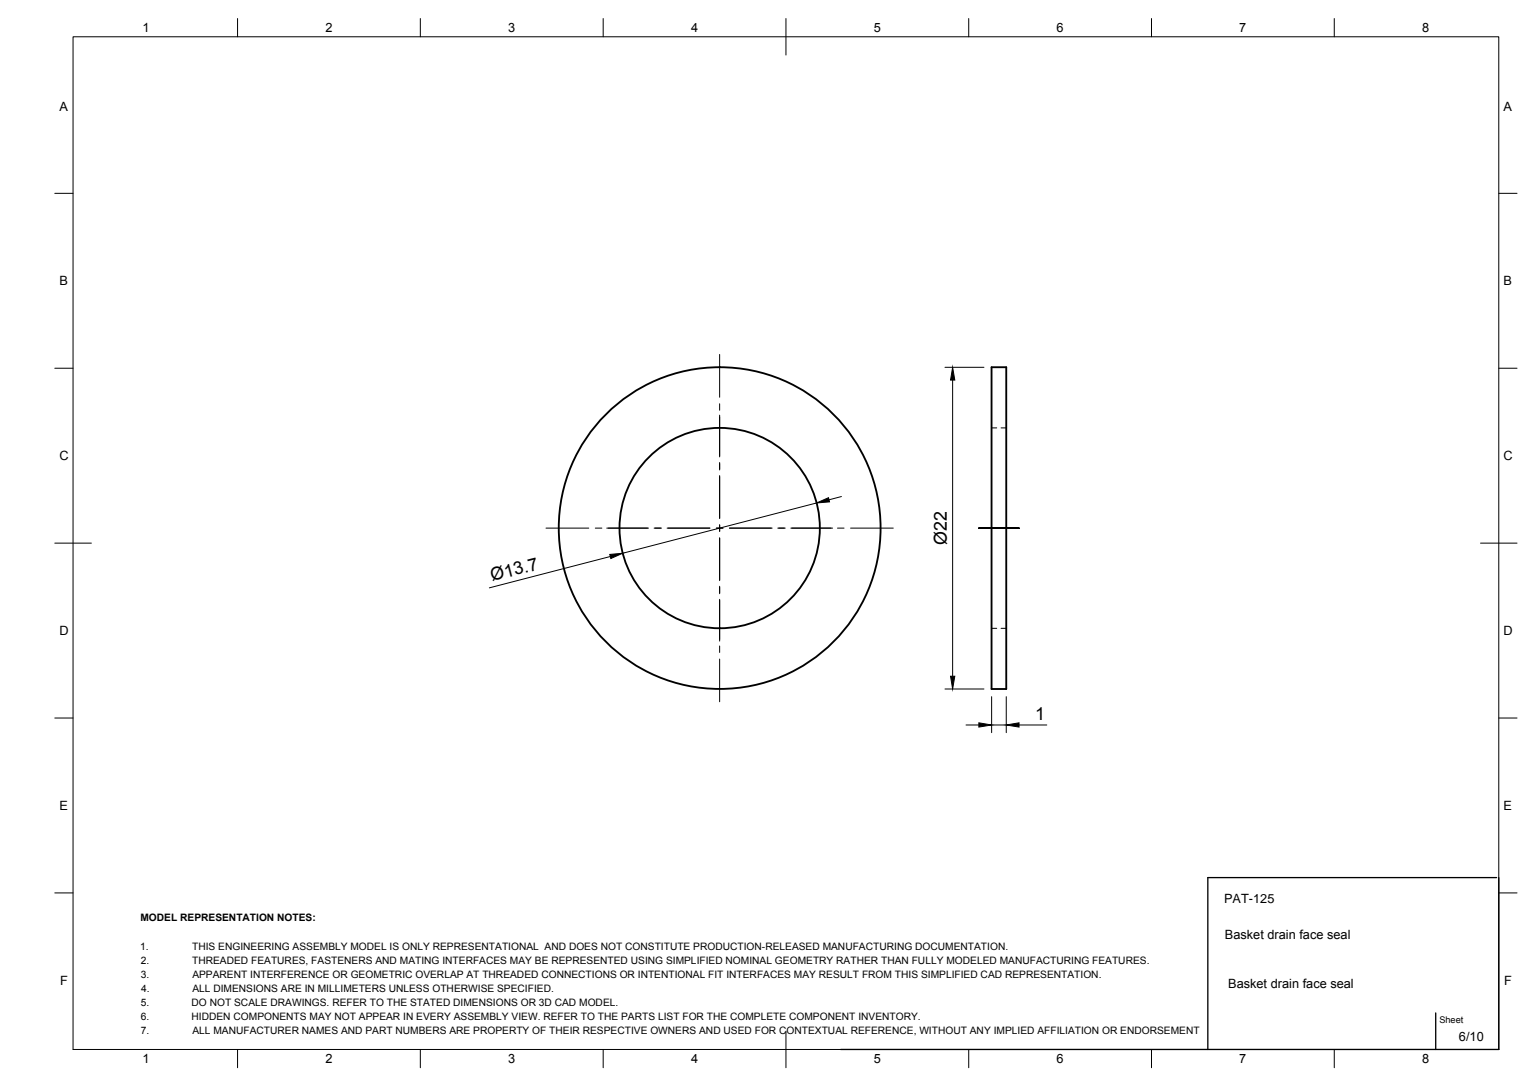
ISO-10303-21;
HEADER;
/* Generated by software containing ST-Developer
 * from STEP Tools, Inc. (www.steptools.com) 
 */

FILE_DESCRIPTION(
/* description */ ('Y-strainer with drain'),
/* implementation_level */ '2;1');

FILE_NAME(
/* name */ 'Basket drain face seal.step',
/* time_stamp */ '2026-10-28T00:41:55-07:00',
/* author */ (''),
/* organization */ (''),
/* preprocessor_version */ 'ST-DEVELOPER v20.2',
/* originating_system */ 'Autodesk Translation Framework v15.17.0.0',
/* authorisation */ '');

FILE_SCHEMA (('AUTOMOTIVE_DESIGN { 1 0 10303 214 3 1 1 }'));
ENDSEC;

DATA;
#10=MECHANICAL_DESIGN_GEOMETRIC_PRESENTATION_REPRESENTATION('',(#96),#8864);
#78=SHAPE_REPRESENTATION_RELATIONSHIP('SRR','None',#8910,#87);
#87=ADVANCED_BREP_SHAPE_REPRESENTATION('',(#105),#8858);
#96=STYLED_ITEM('',(#9040),#105);
#105=MANIFOLD_SOLID_BREP('Body1',#3386);
#427=FACE_BOUND('',#871,.T.);
#428=FACE_BOUND('',#873,.T.);
#483=PLANE('',#3646);
#484=PLANE('',#3647);
#608=FACE_OUTER_BOUND('',#868,.T.);
#609=FACE_OUTER_BOUND('',#869,.T.);
#610=FACE_OUTER_BOUND('',#870,.T.);
#611=FACE_OUTER_BOUND('',#872,.T.);
#868=EDGE_LOOP('',(#2882,#2883,#2884,#2885));
#869=EDGE_LOOP('',(#2886,#2887,#2888,#2889));
#870=EDGE_LOOP('',(#2890));
#871=EDGE_LOOP('',(#2891));
#872=EDGE_LOOP('',(#2892));
#873=EDGE_LOOP('',(#2893));
#1043=LINE('',#8549,#1206);
#1044=LINE('',#8555,#1207);
#1206=VECTOR('',#4151,0.685);
#1207=VECTOR('',#4158,1.1);
#1331=CIRCLE('',#3641,0.685);
#1332=CIRCLE('',#3642,0.685);
#1333=CIRCLE('',#3644,1.1);
#1334=CIRCLE('',#3645,1.1);
#1637=VERTEX_POINT('',#8546);
#1638=VERTEX_POINT('',#8548);
#1639=VERTEX_POINT('',#8552);
#1640=VERTEX_POINT('',#8554);
#2065=EDGE_CURVE('',#1637,#1637,#1331,.T.);
#2066=EDGE_CURVE('',#1637,#1638,#1043,.T.);
#2067=EDGE_CURVE('',#1638,#1638,#1332,.T.);
#2068=EDGE_CURVE('',#1639,#1639,#1333,.T.);
#2069=EDGE_CURVE('',#1639,#1640,#1044,.T.);
#2070=EDGE_CURVE('',#1640,#1640,#1334,.T.);
#2882=ORIENTED_EDGE('',*,*,#2065,.F.);
#2883=ORIENTED_EDGE('',*,*,#2066,.T.);
#2884=ORIENTED_EDGE('',*,*,#2067,.T.);
#2885=ORIENTED_EDGE('',*,*,#2066,.F.);
#2886=ORIENTED_EDGE('',*,*,#2068,.F.);
#2887=ORIENTED_EDGE('',*,*,#2069,.T.);
#2888=ORIENTED_EDGE('',*,*,#2070,.T.);
#2889=ORIENTED_EDGE('',*,*,#2069,.F.);
#2890=ORIENTED_EDGE('',*,*,#2068,.T.);
#2891=ORIENTED_EDGE('',*,*,#2065,.T.);
#2892=ORIENTED_EDGE('',*,*,#2070,.F.);
#2893=ORIENTED_EDGE('',*,*,#2067,.F.);
#3210=CYLINDRICAL_SURFACE('',#3640,0.685);
#3211=CYLINDRICAL_SURFACE('',#3643,1.1);
#3319=ADVANCED_FACE('',(#608),#3210,.F.);
#3320=ADVANCED_FACE('',(#609),#3211,.T.);
#3321=ADVANCED_FACE('',(#610,#427),#483,.T.);
#3322=ADVANCED_FACE('',(#611,#428),#484,.F.);
#3386=CLOSED_SHELL('',(#3319,#3320,#3321,#3322));
#3639=AXIS2_PLACEMENT_3D('',#8544,#4145,#4146);
#3640=AXIS2_PLACEMENT_3D('',#8545,#4147,#4148);
#3641=AXIS2_PLACEMENT_3D('',#8547,#4149,#4150);
#3642=AXIS2_PLACEMENT_3D('',#8550,#4152,#4153);
#3643=AXIS2_PLACEMENT_3D('',#8551,#4154,#4155);
#3644=AXIS2_PLACEMENT_3D('',#8553,#4156,#4157);
#3645=AXIS2_PLACEMENT_3D('',#8556,#4159,#4160);
#3646=AXIS2_PLACEMENT_3D('',#8557,#4161,#4162);
#3647=AXIS2_PLACEMENT_3D('',#8558,#4163,#4164);
#4145=DIRECTION('axis',(0.,0.,1.));
#4146=DIRECTION('refdir',(1.,0.,0.));
#4147=DIRECTION('center_axis',(0.707106781186548,0.,-0.707106781186547));
#4148=DIRECTION('ref_axis',(-0.707106781186547,0.,-0.707106781186548));
#4149=DIRECTION('center_axis',(-0.707106781186548,0.,0.707106781186547));
#4150=DIRECTION('ref_axis',(-0.707106781186547,0.,-0.707106781186548));
#4151=DIRECTION('',(-0.707106781186548,0.,0.707106781186547));
#4152=DIRECTION('center_axis',(-0.707106781186548,0.,0.707106781186547));
#4153=DIRECTION('ref_axis',(-0.707106781186547,0.,-0.707106781186548));
#4154=DIRECTION('center_axis',(0.707106781186548,0.,-0.707106781186547));
#4155=DIRECTION('ref_axis',(-0.707106781186547,0.,-0.707106781186548));
#4156=DIRECTION('center_axis',(0.707106781186548,0.,-0.707106781186547));
#4157=DIRECTION('ref_axis',(-0.707106781186547,0.,-0.707106781186548));
#4158=DIRECTION('',(-0.707106781186548,0.,0.707106781186547));
#4159=DIRECTION('center_axis',(0.707106781186548,0.,-0.707106781186547));
#4160=DIRECTION('ref_axis',(-0.707106781186547,0.,-0.707106781186548));
#4161=DIRECTION('center_axis',(0.707106781186548,0.,-0.707106781186547));
#4162=DIRECTION('ref_axis',(-0.707106781186547,0.,-0.707106781186548));
#4163=DIRECTION('center_axis',(0.707106781186548,0.,-0.707106781186547));
#4164=DIRECTION('ref_axis',(-0.707106781186547,0.,-0.707106781186548));
#8544=CARTESIAN_POINT('',(0.,0.,0.));
#8545=CARTESIAN_POINT('Origin',(3.45477272147525,0.,2.54522727852475));
#8546=CARTESIAN_POINT('',(4.00985154470669,-8.38883057415937E-17,2.95888474551888));
#8547=CARTESIAN_POINT('Origin',(3.5254833995939,0.,2.4745166004061));
#8548=CARTESIAN_POINT('',(3.93914086658804,-8.38883057415937E-17,3.02959542363754));
#8549=CARTESIAN_POINT('',(3.93914086658804,-8.38883057415937E-17,3.02959542363754));
#8550=CARTESIAN_POINT('Origin',(3.45477272147525,0.,2.54522727852475));
#8551=CARTESIAN_POINT('Origin',(3.45477272147525,0.,2.54522727852475));
#8552=CARTESIAN_POINT('',(4.30330085889911,-1.34711147906209E-16,3.2523340597113));
#8553=CARTESIAN_POINT('Origin',(3.5254833995939,0.,2.4745166004061));
#8554=CARTESIAN_POINT('',(4.23259018078045,-1.34711147906209E-16,3.32304473782995));
#8555=CARTESIAN_POINT('',(4.23259018078045,-1.34711147906209E-16,3.32304473782995));
#8556=CARTESIAN_POINT('Origin',(3.45477272147525,0.,2.54522727852475));
#8557=CARTESIAN_POINT('Origin',(3.5254833995939,0.,2.4745166004061));
#8558=CARTESIAN_POINT('Origin',(3.45477272147525,0.,2.54522727852475));
#8846=UNCERTAINTY_MEASURE_WITH_UNIT(LENGTH_MEASURE(0.001),#8865,
'DISTANCE_ACCURACY_VALUE',
'Maximum model space distance between geometric entities at asserted c
onnectivities');
#8852=UNCERTAINTY_MEASURE_WITH_UNIT(LENGTH_MEASURE(0.001),#8865,
'DISTANCE_ACCURACY_VALUE',
'Maximum model space distance between geometric entities at asserted c
onnectivities');
#8858=(
GEOMETRIC_REPRESENTATION_CONTEXT(3)
GLOBAL_UNCERTAINTY_ASSIGNED_CONTEXT((#8846))
GLOBAL_UNIT_ASSIGNED_CONTEXT((#8865,#8867,#8868))
REPRESENTATION_CONTEXT('','3D')
);
#8864=(
GEOMETRIC_REPRESENTATION_CONTEXT(3)
GLOBAL_UNCERTAINTY_ASSIGNED_CONTEXT((#8852))
GLOBAL_UNIT_ASSIGNED_CONTEXT((#8865,#8867,#8868))
REPRESENTATION_CONTEXT('','3D')
);
#8865=(
LENGTH_UNIT()
NAMED_UNIT(*)
SI_UNIT(.CENTI.,.METRE.)
);
#8867=(
NAMED_UNIT(*)
PLANE_ANGLE_UNIT()
SI_UNIT($,.RADIAN.)
);
#8868=(
NAMED_UNIT(*)
SI_UNIT($,.STERADIAN.)
SOLID_ANGLE_UNIT()
);
#8874=SHAPE_DEFINITION_REPRESENTATION(#8885,#8910);
#8885=PRODUCT_DEFINITION_SHAPE('',$,#8922);
#8910=SHAPE_REPRESENTATION('',(#3639),#8858);
#8916=PRODUCT_DEFINITION_CONTEXT('part definition',#8951,'design');
#8922=PRODUCT_DEFINITION('Basket drain face seal',
'Basket drain face seal',#8933,#8916);
#8933=PRODUCT_DEFINITION_FORMATION('',$,#8958);
#8951=APPLICATION_CONTEXT(
'Core Data for Automotive Mechanical Design Process');
#8952=PRODUCT_CONTEXT('part definition',#8951,'mechanical');
#8958=PRODUCT('Basket drain face seal','Basket drain face seal',
'Basket drain face seal',(#8952));
#9034=COLOUR_RGB('Black',0.12,0.14,0.17);
#9035=FILL_AREA_STYLE_COLOUR('',#9034);
#9036=FILL_AREA_STYLE('',(#9035));
#9037=SURFACE_STYLE_FILL_AREA(#9036);
#9038=SURFACE_SIDE_STYLE('',(#9037));
#9039=SURFACE_STYLE_USAGE(.BOTH.,#9038);
#9040=PRESENTATION_STYLE_ASSIGNMENT((#9039));
ENDSEC;
END-ISO-10303-21;
